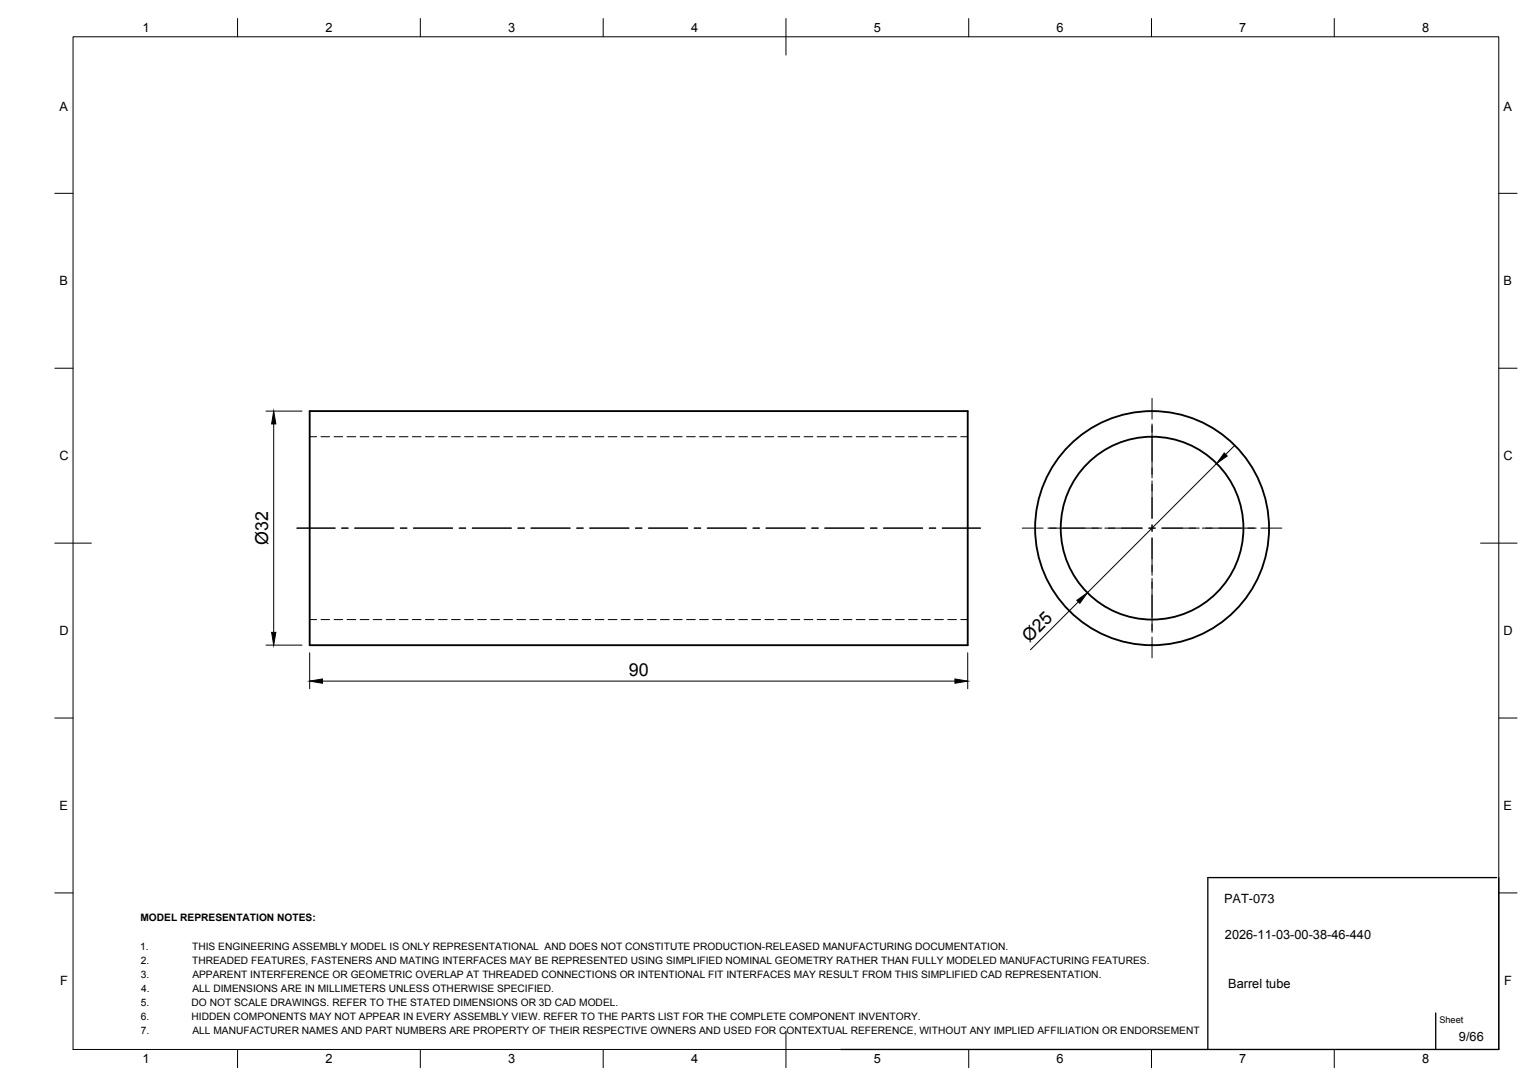
ISO-10303-21;
HEADER;
/* Generated by software containing ST-Developer
 * from STEP Tools, Inc. (www.steptools.com) 
 */

FILE_DESCRIPTION(
/* description */ ('Manual piston pump'),
/* implementation_level */ '2;1');

FILE_NAME(
/* name */ 'Barrel tube.step',
/* time_stamp */ '2026-11-02T16:54:23-08:00',
/* author */ (''),
/* organization */ (''),
/* preprocessor_version */ 'ST-DEVELOPER v20.2',
/* originating_system */ 'Autodesk Translation Framework v15.17.0.0',
/* authorisation */ '');

FILE_SCHEMA (('AUTOMOTIVE_DESIGN { 1 0 10303 214 3 1 1 }'));
ENDSEC;

DATA;
#10=MECHANICAL_DESIGN_GEOMETRIC_PRESENTATION_REPRESENTATION('',(#692),#19043);
#566=SHAPE_REPRESENTATION_RELATIONSHIP('SRR','None',#19312,#629);
#629=ADVANCED_BREP_SHAPE_REPRESENTATION('',(#764),#18979);
#692=STYLED_ITEM('',(#19661),#764);
#764=MANIFOLD_SOLID_BREP('Body1',#9476);
#874=FACE_BOUND('',#1997,.T.);
#875=FACE_BOUND('',#1999,.T.);
#1128=CYLINDRICAL_SURFACE('',#10406,1.25);
#1129=CYLINDRICAL_SURFACE('',#10409,1.6);
#1372=FACE_OUTER_BOUND('',#1994,.T.);
#1373=FACE_OUTER_BOUND('',#1995,.T.);
#1374=FACE_OUTER_BOUND('',#1996,.T.);
#1375=FACE_OUTER_BOUND('',#1998,.T.);
#1994=EDGE_LOOP('',(#6647,#6648,#6649,#6650));
#1995=EDGE_LOOP('',(#6651,#6652,#6653,#6654));
#1996=EDGE_LOOP('',(#6655));
#1997=EDGE_LOOP('',(#6656));
#1998=EDGE_LOOP('',(#6657));
#1999=EDGE_LOOP('',(#6658));
#2739=CIRCLE('',#10407,1.25);
#2740=CIRCLE('',#10408,1.25);
#2741=CIRCLE('',#10410,1.6);
#2742=CIRCLE('',#10411,1.6);
#3255=LINE('',#15056,#3859);
#3256=LINE('',#15062,#3860);
#3859=VECTOR('',#11933,1.25);
#3860=VECTOR('',#11940,1.6);
#4479=VERTEX_POINT('',#15053);
#4480=VERTEX_POINT('',#15055);
#4481=VERTEX_POINT('',#15059);
#4482=VERTEX_POINT('',#15061);
#5310=EDGE_CURVE('',#4479,#4479,#2739,.T.);
#5311=EDGE_CURVE('',#4479,#4480,#3255,.T.);
#5312=EDGE_CURVE('',#4480,#4480,#2740,.T.);
#5313=EDGE_CURVE('',#4481,#4481,#2741,.T.);
#5314=EDGE_CURVE('',#4481,#4482,#3256,.T.);
#5315=EDGE_CURVE('',#4482,#4482,#2742,.T.);
#6647=ORIENTED_EDGE('',*,*,#5310,.F.);
#6648=ORIENTED_EDGE('',*,*,#5311,.T.);
#6649=ORIENTED_EDGE('',*,*,#5312,.T.);
#6650=ORIENTED_EDGE('',*,*,#5311,.F.);
#6651=ORIENTED_EDGE('',*,*,#5313,.F.);
#6652=ORIENTED_EDGE('',*,*,#5314,.T.);
#6653=ORIENTED_EDGE('',*,*,#5315,.T.);
#6654=ORIENTED_EDGE('',*,*,#5314,.F.);
#6655=ORIENTED_EDGE('',*,*,#5313,.T.);
#6656=ORIENTED_EDGE('',*,*,#5310,.T.);
#6657=ORIENTED_EDGE('',*,*,#5315,.F.);
#6658=ORIENTED_EDGE('',*,*,#5312,.F.);
#8616=PLANE('',#10412);
#8617=PLANE('',#10413);
#8977=ADVANCED_FACE('',(#1372),#1128,.F.);
#8978=ADVANCED_FACE('',(#1373),#1129,.T.);
#8979=ADVANCED_FACE('',(#1374,#874),#8616,.T.);
#8980=ADVANCED_FACE('',(#1375,#875),#8617,.F.);
#9476=CLOSED_SHELL('',(#8977,#8978,#8979,#8980));
#10405=AXIS2_PLACEMENT_3D('',#15051,#11927,#11928);
#10406=AXIS2_PLACEMENT_3D('',#15052,#11929,#11930);
#10407=AXIS2_PLACEMENT_3D('',#15054,#11931,#11932);
#10408=AXIS2_PLACEMENT_3D('',#15057,#11934,#11935);
#10409=AXIS2_PLACEMENT_3D('',#15058,#11936,#11937);
#10410=AXIS2_PLACEMENT_3D('',#15060,#11938,#11939);
#10411=AXIS2_PLACEMENT_3D('',#15063,#11941,#11942);
#10412=AXIS2_PLACEMENT_3D('',#15064,#11943,#11944);
#10413=AXIS2_PLACEMENT_3D('',#15065,#11945,#11946);
#11927=DIRECTION('axis',(0.,0.,1.));
#11928=DIRECTION('refdir',(1.,0.,0.));
#11929=DIRECTION('center_axis',(0.,1.,0.));
#11930=DIRECTION('ref_axis',(1.,0.,0.));
#11931=DIRECTION('center_axis',(0.,-1.,0.));
#11932=DIRECTION('ref_axis',(1.,0.,0.));
#11933=DIRECTION('',(0.,-1.,0.));
#11934=DIRECTION('center_axis',(0.,-1.,0.));
#11935=DIRECTION('ref_axis',(1.,0.,0.));
#11936=DIRECTION('center_axis',(0.,1.,0.));
#11937=DIRECTION('ref_axis',(1.,0.,0.));
#11938=DIRECTION('center_axis',(0.,1.,0.));
#11939=DIRECTION('ref_axis',(1.,0.,0.));
#11940=DIRECTION('',(0.,-1.,0.));
#11941=DIRECTION('center_axis',(0.,1.,0.));
#11942=DIRECTION('ref_axis',(1.,0.,0.));
#11943=DIRECTION('center_axis',(0.,1.,0.));
#11944=DIRECTION('ref_axis',(1.,0.,0.));
#11945=DIRECTION('center_axis',(0.,1.,0.));
#11946=DIRECTION('ref_axis',(1.,0.,0.));
#15051=CARTESIAN_POINT('',(0.,0.,0.));
#15052=CARTESIAN_POINT('Origin',(0.,1.8,4.5));
#15053=CARTESIAN_POINT('',(-1.25,10.8,4.5));
#15054=CARTESIAN_POINT('Origin',(0.,10.8,4.5));
#15055=CARTESIAN_POINT('',(-1.25,1.8,4.5));
#15056=CARTESIAN_POINT('',(-1.25,1.8,4.5));
#15057=CARTESIAN_POINT('Origin',(0.,1.8,4.5));
#15058=CARTESIAN_POINT('Origin',(0.,1.8,4.5));
#15059=CARTESIAN_POINT('',(-1.6,10.8,4.5));
#15060=CARTESIAN_POINT('Origin',(0.,10.8,4.5));
#15061=CARTESIAN_POINT('',(-1.6,1.8,4.5));
#15062=CARTESIAN_POINT('',(-1.6,1.8,4.5));
#15063=CARTESIAN_POINT('Origin',(0.,1.8,4.5));
#15064=CARTESIAN_POINT('Origin',(0.,10.8,4.5));
#15065=CARTESIAN_POINT('Origin',(0.,1.8,4.5));
#18908=UNCERTAINTY_MEASURE_WITH_UNIT(LENGTH_MEASURE(0.001),#19044,
'DISTANCE_ACCURACY_VALUE',
'Maximum model space distance between geometric entities at asserted c
onnectivities');
#18972=UNCERTAINTY_MEASURE_WITH_UNIT(LENGTH_MEASURE(0.001),#19044,
'DISTANCE_ACCURACY_VALUE',
'Maximum model space distance between geometric entities at asserted c
onnectivities');
#18979=(
GEOMETRIC_REPRESENTATION_CONTEXT(3)
GLOBAL_UNCERTAINTY_ASSIGNED_CONTEXT((#18908))
GLOBAL_UNIT_ASSIGNED_CONTEXT((#19044,#19046,#19047))
REPRESENTATION_CONTEXT('','3D')
);
#19043=(
GEOMETRIC_REPRESENTATION_CONTEXT(3)
GLOBAL_UNCERTAINTY_ASSIGNED_CONTEXT((#18972))
GLOBAL_UNIT_ASSIGNED_CONTEXT((#19044,#19046,#19047))
REPRESENTATION_CONTEXT('','3D')
);
#19044=(
LENGTH_UNIT()
NAMED_UNIT(*)
SI_UNIT(.CENTI.,.METRE.)
);
#19046=(
NAMED_UNIT(*)
PLANE_ANGLE_UNIT()
SI_UNIT($,.RADIAN.)
);
#19047=(
NAMED_UNIT(*)
SI_UNIT($,.STERADIAN.)
SOLID_ANGLE_UNIT()
);
#19054=SHAPE_DEFINITION_REPRESENTATION(#19124,#19312);
#19124=PRODUCT_DEFINITION_SHAPE('',$,#19383);
#19312=SHAPE_REPRESENTATION('',(#10405),#18979);
#19376=PRODUCT_DEFINITION_CONTEXT('part definition',#19588,'design');
#19383=PRODUCT_DEFINITION('2026-11-03-00-38-46-440','Barrel tube',#19453,
#19376);
#19453=PRODUCT_DEFINITION_FORMATION('',$,#19596);
#19588=APPLICATION_CONTEXT(
'Core Data for Automotive Mechanical Design Process');
#19589=PRODUCT_CONTEXT('part definition',#19588,'mechanical');
#19596=PRODUCT('2026-11-03-00-38-46-440','Barrel tube','Barrel tube',(#19589));
#19661=PRESENTATION_STYLE_ASSIGNMENT((#19667));
#19667=SURFACE_STYLE_USAGE(.BOTH.,#19673);
#19673=SURFACE_SIDE_STYLE('',(#19679));
#19679=SURFACE_STYLE_FILL_AREA(#19685);
#19685=FILL_AREA_STYLE('CAD Library Painted - Engineering blue',(#19691));
#19691=FILL_AREA_STYLE_COLOUR('CAD Library Painted - Engineering blue',
#19697);
#19697=COLOUR_RGB('CAD Library Painted - Engineering blue',0.12156862745098,
0.356862745098039,0.6);
ENDSEC;
END-ISO-10303-21;
